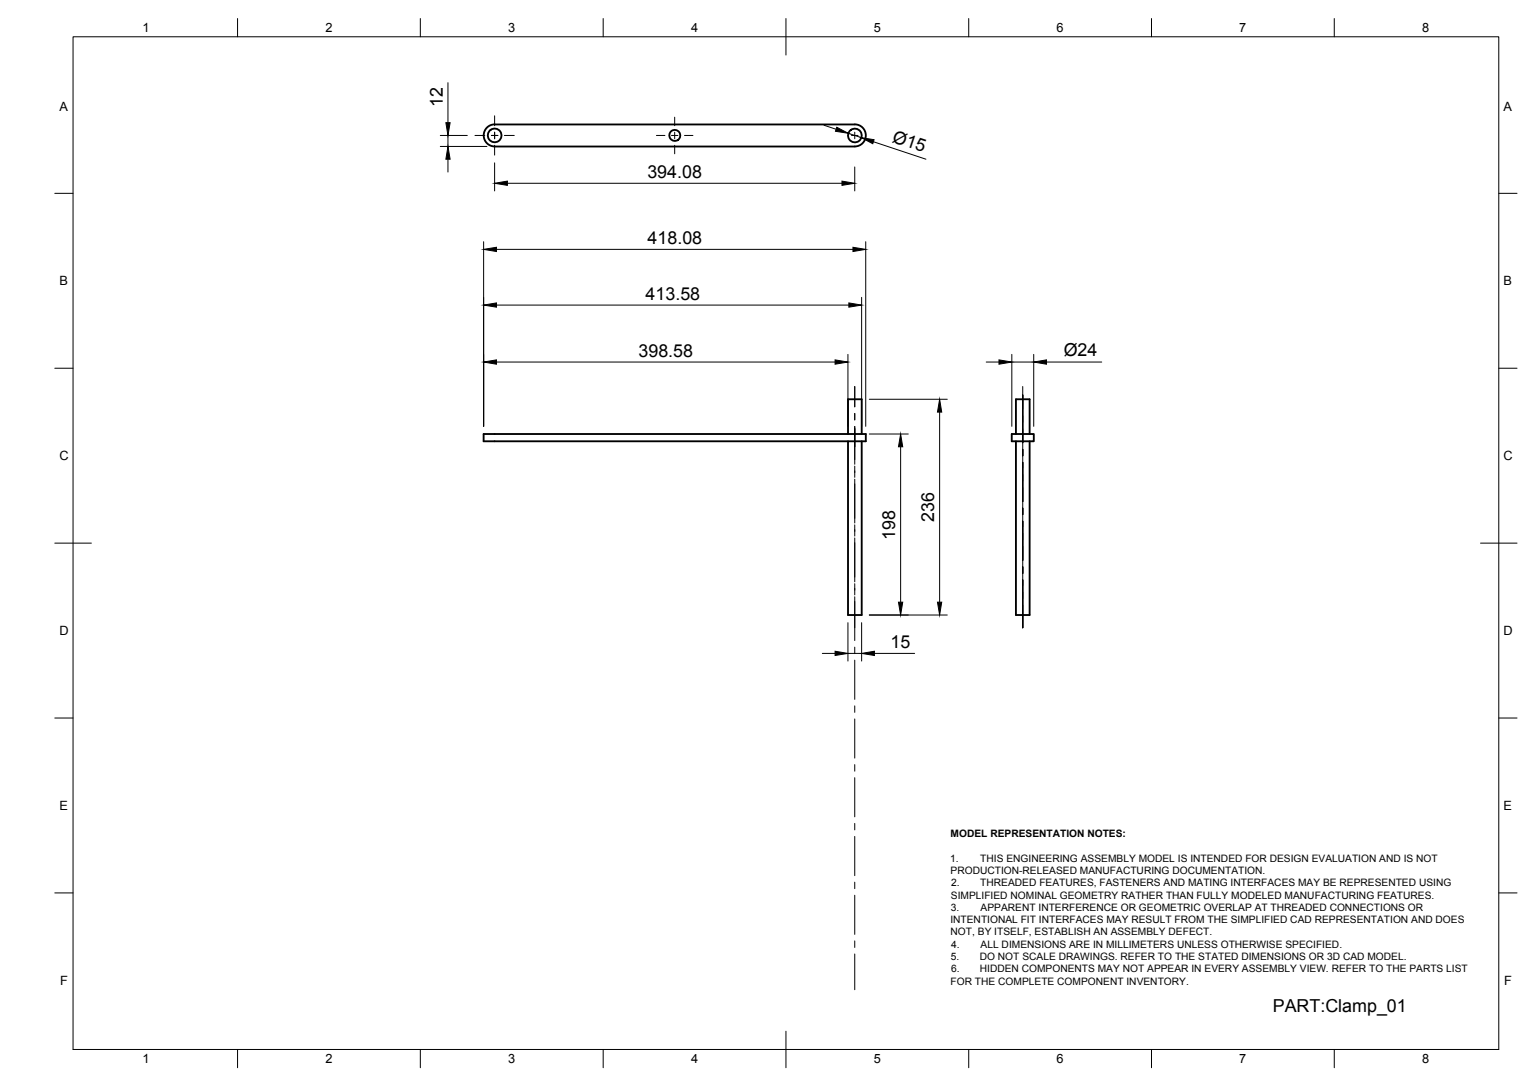
ISO-10303-21;
HEADER;
/* Generated by software containing ST-Developer
 * from STEP Tools, Inc. (www.steptools.com) 
 */

FILE_DESCRIPTION(
/* description */ (''),
/* implementation_level */ '2;1');

FILE_NAME(
/* name */ 'Clamp_01.step',
/* time_stamp */ '2026-10-05T15:35:09-07:00',
/* author */ (''),
/* organization */ (''),
/* preprocessor_version */ 'ST-DEVELOPER v20.2',
/* originating_system */ 'Autodesk Translation Framework v15.15.0.0',
/* authorisation */ '');

FILE_SCHEMA (('AUTOMOTIVE_DESIGN { 1 0 10303 214 3 1 1 }'));
ENDSEC;

DATA;
#10=MECHANICAL_DESIGN_GEOMETRIC_PRESENTATION_REPRESENTATION('',(#546),#74523);
#528=SHAPE_REPRESENTATION_RELATIONSHIP('SRR','None',#74561,#537);
#537=ADVANCED_BREP_SHAPE_REPRESENTATION('',(#555),#74517);
#546=STYLED_ITEM('',(#74612),#555);
#555=MANIFOLD_SOLID_BREP('Body1',#4725);
#581=FACE_BOUND('',#905,.T.);
#582=FACE_BOUND('',#906,.T.);
#583=FACE_BOUND('',#907,.T.);
#584=FACE_BOUND('',#909,.T.);
#585=FACE_BOUND('',#910,.T.);
#586=FACE_BOUND('',#911,.T.);
#637=PLANE('',#4942);
#638=PLANE('',#4946);
#639=PLANE('',#4950);
#640=PLANE('',#4952);
#641=PLANE('',#4956);
#642=PLANE('',#4959);
#734=FACE_OUTER_BOUND('',#898,.T.);
#735=FACE_OUTER_BOUND('',#899,.T.);
#736=FACE_OUTER_BOUND('',#900,.T.);
#737=FACE_OUTER_BOUND('',#901,.T.);
#738=FACE_OUTER_BOUND('',#902,.T.);
#739=FACE_OUTER_BOUND('',#903,.T.);
#740=FACE_OUTER_BOUND('',#904,.T.);
#741=FACE_OUTER_BOUND('',#908,.T.);
#742=FACE_OUTER_BOUND('',#912,.T.);
#743=FACE_OUTER_BOUND('',#913,.T.);
#744=FACE_OUTER_BOUND('',#914,.T.);
#745=FACE_OUTER_BOUND('',#915,.T.);
#898=EDGE_LOOP('',(#3222,#3223,#3224,#3225));
#899=EDGE_LOOP('',(#3226,#3227,#3228,#3229));
#900=EDGE_LOOP('',(#3230,#3231,#3232,#3233));
#901=EDGE_LOOP('',(#3234,#3235,#3236,#3237));
#902=EDGE_LOOP('',(#3238,#3239,#3240,#3241));
#903=EDGE_LOOP('',(#3242,#3243,#3244,#3245));
#904=EDGE_LOOP('',(#3246,#3247,#3248,#3249));
#905=EDGE_LOOP('',(#3250));
#906=EDGE_LOOP('',(#3251));
#907=EDGE_LOOP('',(#3252));
#908=EDGE_LOOP('',(#3253,#3254,#3255,#3256));
#909=EDGE_LOOP('',(#3257));
#910=EDGE_LOOP('',(#3258));
#911=EDGE_LOOP('',(#3259));
#912=EDGE_LOOP('',(#3260,#3261,#3262,#3263));
#913=EDGE_LOOP('',(#3264));
#914=EDGE_LOOP('',(#3265,#3266,#3267,#3268));
#915=EDGE_LOOP('',(#3269));
#1102=LINE('',#6110,#1299);
#1103=LINE('',#6116,#1300);
#1104=LINE('',#6121,#1301);
#1105=LINE('',#6123,#1302);
#1106=LINE('',#6125,#1303);
#1107=LINE('',#6126,#1304);
#1108=LINE('',#6131,#1305);
#1109=LINE('',#6135,#1306);
#1110=LINE('',#6137,#1307);
#1111=LINE('',#6138,#1308);
#1112=LINE('',#6151,#1309);
#1113=LINE('',#6156,#1310);
#1299=VECTOR('',#5396,6.00000000000001);
#1300=VECTOR('',#5403,7.5);
#1301=VECTOR('',#5408,10.);
#1302=VECTOR('',#5409,10.);
#1303=VECTOR('',#5410,10.);
#1304=VECTOR('',#5411,10.);
#1305=VECTOR('',#5416,10.);
#1306=VECTOR('',#5421,10.);
#1307=VECTOR('',#5422,10.);
#1308=VECTOR('',#5423,10.);
#1309=VECTOR('',#5442,7.5);
#1310=VECTOR('',#5449,7.5);
#1460=CIRCLE('',#4937,6.00000000000001);
#1461=CIRCLE('',#4938,6.00000000000001);
#1462=CIRCLE('',#4940,7.5);
#1463=CIRCLE('',#4941,7.5);
#1464=CIRCLE('',#4944,12.);
#1465=CIRCLE('',#4945,12.);
#1466=CIRCLE('',#4948,12.);
#1467=CIRCLE('',#4949,12.);
#1468=CIRCLE('',#4951,7.5);
#1469=CIRCLE('',#4953,7.5);
#1470=CIRCLE('',#4955,7.5);
#1471=CIRCLE('',#4957,7.5);
#1610=VERTEX_POINT('',#6107);
#1611=VERTEX_POINT('',#6109);
#1612=VERTEX_POINT('',#6113);
#1613=VERTEX_POINT('',#6115);
#1614=VERTEX_POINT('',#6119);
#1615=VERTEX_POINT('',#6120);
#1616=VERTEX_POINT('',#6122);
#1617=VERTEX_POINT('',#6124);
#1618=VERTEX_POINT('',#6128);
#1619=VERTEX_POINT('',#6130);
#1620=VERTEX_POINT('',#6134);
#1621=VERTEX_POINT('',#6136);
#1622=VERTEX_POINT('',#6143);
#1623=VERTEX_POINT('',#6146);
#1624=VERTEX_POINT('',#6149);
#1625=VERTEX_POINT('',#6153);
#2312=EDGE_CURVE('',#1610,#1610,#1460,.T.);
#2313=EDGE_CURVE('',#1610,#1611,#1102,.T.);
#2314=EDGE_CURVE('',#1611,#1611,#1461,.T.);
#2315=EDGE_CURVE('',#1612,#1612,#1462,.T.);
#2316=EDGE_CURVE('',#1612,#1613,#1103,.T.);
#2317=EDGE_CURVE('',#1613,#1613,#1463,.T.);
#2318=EDGE_CURVE('',#1614,#1615,#1104,.T.);
#2319=EDGE_CURVE('',#1614,#1616,#1105,.T.);
#2320=EDGE_CURVE('',#1616,#1617,#1106,.T.);
#2321=EDGE_CURVE('',#1615,#1617,#1107,.T.);
#2322=EDGE_CURVE('',#1618,#1614,#1464,.T.);
#2323=EDGE_CURVE('',#1618,#1619,#1108,.T.);
#2324=EDGE_CURVE('',#1619,#1616,#1465,.T.);
#2325=EDGE_CURVE('',#1620,#1618,#1109,.T.);
#2326=EDGE_CURVE('',#1620,#1621,#1110,.T.);
#2327=EDGE_CURVE('',#1621,#1619,#1111,.T.);
#2328=EDGE_CURVE('',#1615,#1620,#1466,.T.);
#2329=EDGE_CURVE('',#1617,#1621,#1467,.T.);
#2330=EDGE_CURVE('',#1622,#1622,#1468,.T.);
#2331=EDGE_CURVE('',#1623,#1623,#1469,.T.);
#2332=EDGE_CURVE('',#1624,#1624,#1470,.T.);
#2333=EDGE_CURVE('',#1624,#1623,#1112,.T.);
#2334=EDGE_CURVE('',#1625,#1625,#1471,.T.);
#2335=EDGE_CURVE('',#1622,#1625,#1113,.T.);
#3222=ORIENTED_EDGE('',*,*,#2312,.F.);
#3223=ORIENTED_EDGE('',*,*,#2313,.T.);
#3224=ORIENTED_EDGE('',*,*,#2314,.F.);
#3225=ORIENTED_EDGE('',*,*,#2313,.F.);
#3226=ORIENTED_EDGE('',*,*,#2315,.T.);
#3227=ORIENTED_EDGE('',*,*,#2316,.T.);
#3228=ORIENTED_EDGE('',*,*,#2317,.F.);
#3229=ORIENTED_EDGE('',*,*,#2316,.F.);
#3230=ORIENTED_EDGE('',*,*,#2318,.F.);
#3231=ORIENTED_EDGE('',*,*,#2319,.T.);
#3232=ORIENTED_EDGE('',*,*,#2320,.T.);
#3233=ORIENTED_EDGE('',*,*,#2321,.F.);
#3234=ORIENTED_EDGE('',*,*,#2322,.F.);
#3235=ORIENTED_EDGE('',*,*,#2323,.T.);
#3236=ORIENTED_EDGE('',*,*,#2324,.T.);
#3237=ORIENTED_EDGE('',*,*,#2319,.F.);
#3238=ORIENTED_EDGE('',*,*,#2325,.F.);
#3239=ORIENTED_EDGE('',*,*,#2326,.T.);
#3240=ORIENTED_EDGE('',*,*,#2327,.T.);
#3241=ORIENTED_EDGE('',*,*,#2323,.F.);
#3242=ORIENTED_EDGE('',*,*,#2328,.F.);
#3243=ORIENTED_EDGE('',*,*,#2321,.T.);
#3244=ORIENTED_EDGE('',*,*,#2329,.T.);
#3245=ORIENTED_EDGE('',*,*,#2326,.F.);
#3246=ORIENTED_EDGE('',*,*,#2329,.F.);
#3247=ORIENTED_EDGE('',*,*,#2320,.F.);
#3248=ORIENTED_EDGE('',*,*,#2324,.F.);
#3249=ORIENTED_EDGE('',*,*,#2327,.F.);
#3250=ORIENTED_EDGE('',*,*,#2312,.T.);
#3251=ORIENTED_EDGE('',*,*,#2315,.F.);
#3252=ORIENTED_EDGE('',*,*,#2330,.F.);
#3253=ORIENTED_EDGE('',*,*,#2328,.T.);
#3254=ORIENTED_EDGE('',*,*,#2325,.T.);
#3255=ORIENTED_EDGE('',*,*,#2322,.T.);
#3256=ORIENTED_EDGE('',*,*,#2318,.T.);
#3257=ORIENTED_EDGE('',*,*,#2314,.T.);
#3258=ORIENTED_EDGE('',*,*,#2317,.T.);
#3259=ORIENTED_EDGE('',*,*,#2331,.F.);
#3260=ORIENTED_EDGE('',*,*,#2332,.F.);
#3261=ORIENTED_EDGE('',*,*,#2333,.T.);
#3262=ORIENTED_EDGE('',*,*,#2331,.T.);
#3263=ORIENTED_EDGE('',*,*,#2333,.F.);
#3264=ORIENTED_EDGE('',*,*,#2334,.T.);
#3265=ORIENTED_EDGE('',*,*,#2330,.T.);
#3266=ORIENTED_EDGE('',*,*,#2335,.T.);
#3267=ORIENTED_EDGE('',*,*,#2334,.F.);
#3268=ORIENTED_EDGE('',*,*,#2335,.F.);
#3269=ORIENTED_EDGE('',*,*,#2332,.T.);
#4538=CYLINDRICAL_SURFACE('',#4936,6.00000000000001);
#4539=CYLINDRICAL_SURFACE('',#4939,7.5);
#4540=CYLINDRICAL_SURFACE('',#4943,12.);
#4541=CYLINDRICAL_SURFACE('',#4947,12.);
#4542=CYLINDRICAL_SURFACE('',#4954,7.5);
#4543=CYLINDRICAL_SURFACE('',#4958,7.5);
#4630=ADVANCED_FACE('',(#734),#4538,.F.);
#4631=ADVANCED_FACE('',(#735),#4539,.F.);
#4632=ADVANCED_FACE('',(#736),#637,.F.);
#4633=ADVANCED_FACE('',(#737),#4540,.T.);
#4634=ADVANCED_FACE('',(#738),#638,.F.);
#4635=ADVANCED_FACE('',(#739),#4541,.T.);
#4636=ADVANCED_FACE('',(#740,#581,#582,#583),#639,.F.);
#4637=ADVANCED_FACE('',(#741,#584,#585,#586),#640,.T.);
#4638=ADVANCED_FACE('',(#742),#4542,.T.);
#4639=ADVANCED_FACE('',(#743),#641,.F.);
#4640=ADVANCED_FACE('',(#744),#4543,.T.);
#4641=ADVANCED_FACE('',(#745),#642,.T.);
#4725=CLOSED_SHELL('',(#4630,#4631,#4632,#4633,#4634,#4635,#4636,#4637,
#4638,#4639,#4640,#4641));
#4935=AXIS2_PLACEMENT_3D('',#6105,#5390,#5391);
#4936=AXIS2_PLACEMENT_3D('',#6106,#5392,#5393);
#4937=AXIS2_PLACEMENT_3D('',#6108,#5394,#5395);
#4938=AXIS2_PLACEMENT_3D('',#6111,#5397,#5398);
#4939=AXIS2_PLACEMENT_3D('',#6112,#5399,#5400);
#4940=AXIS2_PLACEMENT_3D('',#6114,#5401,#5402);
#4941=AXIS2_PLACEMENT_3D('',#6117,#5404,#5405);
#4942=AXIS2_PLACEMENT_3D('',#6118,#5406,#5407);
#4943=AXIS2_PLACEMENT_3D('',#6127,#5412,#5413);
#4944=AXIS2_PLACEMENT_3D('',#6129,#5414,#5415);
#4945=AXIS2_PLACEMENT_3D('',#6132,#5417,#5418);
#4946=AXIS2_PLACEMENT_3D('',#6133,#5419,#5420);
#4947=AXIS2_PLACEMENT_3D('',#6139,#5424,#5425);
#4948=AXIS2_PLACEMENT_3D('',#6140,#5426,#5427);
#4949=AXIS2_PLACEMENT_3D('',#6141,#5428,#5429);
#4950=AXIS2_PLACEMENT_3D('',#6142,#5430,#5431);
#4951=AXIS2_PLACEMENT_3D('',#6144,#5432,#5433);
#4952=AXIS2_PLACEMENT_3D('',#6145,#5434,#5435);
#4953=AXIS2_PLACEMENT_3D('',#6147,#5436,#5437);
#4954=AXIS2_PLACEMENT_3D('',#6148,#5438,#5439);
#4955=AXIS2_PLACEMENT_3D('',#6150,#5440,#5441);
#4956=AXIS2_PLACEMENT_3D('',#6152,#5443,#5444);
#4957=AXIS2_PLACEMENT_3D('',#6154,#5445,#5446);
#4958=AXIS2_PLACEMENT_3D('',#6155,#5447,#5448);
#4959=AXIS2_PLACEMENT_3D('',#6157,#5450,#5451);
#5390=DIRECTION('axis',(0.,0.,1.));
#5391=DIRECTION('refdir',(1.,0.,0.));
#5392=DIRECTION('center_axis',(0.,1.,0.));
#5393=DIRECTION('ref_axis',(1.,0.,0.));
#5394=DIRECTION('center_axis',(0.,1.,0.));
#5395=DIRECTION('ref_axis',(1.,0.,0.));
#5396=DIRECTION('',(0.,1.,0.));
#5397=DIRECTION('center_axis',(0.,-1.,0.));
#5398=DIRECTION('ref_axis',(1.,0.,0.));
#5399=DIRECTION('center_axis',(0.,1.,0.));
#5400=DIRECTION('ref_axis',(1.,0.,0.));
#5401=DIRECTION('center_axis',(0.,-1.,0.));
#5402=DIRECTION('ref_axis',(1.,0.,0.));
#5403=DIRECTION('',(0.,1.,0.));
#5404=DIRECTION('center_axis',(0.,-1.,0.));
#5405=DIRECTION('ref_axis',(1.,0.,0.));
#5406=DIRECTION('center_axis',(0.812015371342714,0.,-0.583636048152575));
#5407=DIRECTION('ref_axis',(0.583636048152575,0.,0.812015371342714));
#5408=DIRECTION('',(0.583636048152575,0.,0.812015371342714));
#5409=DIRECTION('',(0.,-1.,0.));
#5410=DIRECTION('',(0.583636048152575,0.,0.812015371342714));
#5411=DIRECTION('',(0.,-1.,0.));
#5412=DIRECTION('center_axis',(0.,1.,0.));
#5413=DIRECTION('ref_axis',(0.812015371342714,0.,-0.583636048152574));
#5414=DIRECTION('center_axis',(0.,1.,0.));
#5415=DIRECTION('ref_axis',(0.812015371342714,0.,-0.583636048152574));
#5416=DIRECTION('',(0.,-1.,0.));
#5417=DIRECTION('center_axis',(0.,1.,0.));
#5418=DIRECTION('ref_axis',(0.812015371342714,0.,-0.583636048152574));
#5419=DIRECTION('center_axis',(-0.812015371342714,0.,0.583636048152575));
#5420=DIRECTION('ref_axis',(-0.583636048152575,0.,-0.812015371342714));
#5421=DIRECTION('',(-0.583636048152575,0.,-0.812015371342714));
#5422=DIRECTION('',(0.,-1.,0.));
#5423=DIRECTION('',(-0.583636048152575,0.,-0.812015371342714));
#5424=DIRECTION('center_axis',(0.,1.,0.));
#5425=DIRECTION('ref_axis',(-0.812015371342714,0.,0.583636048152574));
#5426=DIRECTION('center_axis',(0.,1.,0.));
#5427=DIRECTION('ref_axis',(-0.812015371342714,0.,0.583636048152574));
#5428=DIRECTION('center_axis',(0.,1.,0.));
#5429=DIRECTION('ref_axis',(-0.812015371342714,0.,0.583636048152574));
#5430=DIRECTION('center_axis',(0.,1.,0.));
#5431=DIRECTION('ref_axis',(1.,0.,0.));
#5432=DIRECTION('center_axis',(0.,-1.,0.));
#5433=DIRECTION('ref_axis',(1.,0.,0.));
#5434=DIRECTION('center_axis',(0.,1.,0.));
#5435=DIRECTION('ref_axis',(1.,0.,0.));
#5436=DIRECTION('center_axis',(0.,1.,0.));
#5437=DIRECTION('ref_axis',(1.,0.,0.));
#5438=DIRECTION('center_axis',(0.,1.,0.));
#5439=DIRECTION('ref_axis',(1.,0.,0.));
#5440=DIRECTION('center_axis',(0.,1.,0.));
#5441=DIRECTION('ref_axis',(1.,0.,0.));
#5442=DIRECTION('',(0.,-1.,0.));
#5443=DIRECTION('center_axis',(0.,1.,0.));
#5444=DIRECTION('ref_axis',(1.,0.,0.));
#5445=DIRECTION('center_axis',(0.,-1.,0.));
#5446=DIRECTION('ref_axis',(1.,0.,0.));
#5447=DIRECTION('center_axis',(0.,1.,0.));
#5448=DIRECTION('ref_axis',(1.,0.,0.));
#5449=DIRECTION('',(0.,-1.,0.));
#5450=DIRECTION('center_axis',(0.,1.,0.));
#5451=DIRECTION('ref_axis',(1.,0.,0.));
#6105=CARTESIAN_POINT('',(0.,0.,0.));
#6106=CARTESIAN_POINT('Origin',(60.231676812499,95.,175.));
#6107=CARTESIAN_POINT('',(54.231676812499,72.,175.));
#6108=CARTESIAN_POINT('Origin',(60.231676812499,72.,175.));
#6109=CARTESIAN_POINT('',(54.231676812499,80.,175.));
#6110=CARTESIAN_POINT('',(54.231676812499,95.,175.));
#6111=CARTESIAN_POINT('Origin',(60.231676812499,80.,175.));
#6112=CARTESIAN_POINT('Origin',(175.231676812499,80.,335.));
#6113=CARTESIAN_POINT('',(167.731676812499,72.,335.));
#6114=CARTESIAN_POINT('Origin',(175.231676812499,72.,335.));
#6115=CARTESIAN_POINT('',(167.731676812499,80.,335.));
#6116=CARTESIAN_POINT('',(167.731676812499,80.,335.));
#6117=CARTESIAN_POINT('Origin',(175.231676812499,80.,335.));
#6118=CARTESIAN_POINT('Origin',(-64.5125076436135,80.,22.0036325778309));
#6119=CARTESIAN_POINT('',(-64.5125076436135,80.,22.0036325778309));
#6120=CARTESIAN_POINT('',(165.487492356386,80.,342.003632577831));
#6121=CARTESIAN_POINT('',(-64.5125076436135,80.,22.0036325778309));
#6122=CARTESIAN_POINT('',(-64.5125076436135,72.,22.0036325778309));
#6123=CARTESIAN_POINT('',(-64.5125076436135,80.,22.0036325778309));
#6124=CARTESIAN_POINT('',(165.487492356386,72.,342.003632577831));
#6125=CARTESIAN_POINT('',(-64.5125076436135,72.,22.0036325778309));
#6126=CARTESIAN_POINT('',(165.487492356386,80.,342.003632577831));
#6127=CARTESIAN_POINT('Origin',(-54.7683231875009,80.,15.));
#6128=CARTESIAN_POINT('',(-45.0241387313884,80.,7.99636742216912));
#6129=CARTESIAN_POINT('Origin',(-54.7683231875009,80.,15.));
#6130=CARTESIAN_POINT('',(-45.0241387313884,72.,7.99636742216912));
#6131=CARTESIAN_POINT('',(-45.0241387313884,80.,7.99636742216912));
#6132=CARTESIAN_POINT('Origin',(-54.7683231875009,72.,15.));
#6133=CARTESIAN_POINT('Origin',(184.975861268612,80.,327.996367422169));
#6134=CARTESIAN_POINT('',(184.975861268612,80.,327.996367422169));
#6135=CARTESIAN_POINT('',(184.975861268612,80.,327.996367422169));
#6136=CARTESIAN_POINT('',(184.975861268612,72.,327.996367422169));
#6137=CARTESIAN_POINT('',(184.975861268612,80.,327.996367422169));
#6138=CARTESIAN_POINT('',(184.975861268612,72.,327.996367422169));
#6139=CARTESIAN_POINT('Origin',(175.231676812499,80.,335.));
#6140=CARTESIAN_POINT('Origin',(175.231676812499,80.,335.));
#6141=CARTESIAN_POINT('Origin',(175.231676812499,72.,335.));
#6142=CARTESIAN_POINT('Origin',(60.231676812499,72.,175.));
#6143=CARTESIAN_POINT('',(-62.2683231875009,72.,15.));
#6144=CARTESIAN_POINT('Origin',(-54.7683231875009,72.,15.));
#6145=CARTESIAN_POINT('Origin',(60.231676812499,80.,175.));
#6146=CARTESIAN_POINT('',(-62.2683231875009,80.,15.));
#6147=CARTESIAN_POINT('Origin',(-54.7683231875009,80.,15.));
#6148=CARTESIAN_POINT('Origin',(-54.7683231875009,0.,15.));
#6149=CARTESIAN_POINT('',(-62.2683231875009,118.,15.));
#6150=CARTESIAN_POINT('Origin',(-54.7683231875009,118.,15.));
#6151=CARTESIAN_POINT('',(-62.2683231875009,0.,15.));
#6152=CARTESIAN_POINT('Origin',(-54.7683231875009,-118.,15.));
#6153=CARTESIAN_POINT('',(-62.2683231875009,-118.,15.));
#6154=CARTESIAN_POINT('Origin',(-54.7683231875009,-118.,15.));
#6155=CARTESIAN_POINT('Origin',(-54.7683231875009,0.,15.));
#6156=CARTESIAN_POINT('',(-62.2683231875009,0.,15.));
#6157=CARTESIAN_POINT('Origin',(-54.7683231875009,118.,15.));
#74506=UNCERTAINTY_MEASURE_WITH_UNIT(LENGTH_MEASURE(0.01),#74524,
'DISTANCE_ACCURACY_VALUE',
'Maximum model space distance between geometric entities at asserted c
onnectivities');
#74512=UNCERTAINTY_MEASURE_WITH_UNIT(LENGTH_MEASURE(0.01),#74524,
'DISTANCE_ACCURACY_VALUE',
'Maximum model space distance between geometric entities at asserted c
onnectivities');
#74517=(
GEOMETRIC_REPRESENTATION_CONTEXT(3)
GLOBAL_UNCERTAINTY_ASSIGNED_CONTEXT((#74506))
GLOBAL_UNIT_ASSIGNED_CONTEXT((#74524,#74526,#74527))
REPRESENTATION_CONTEXT('','3D')
);
#74523=(
GEOMETRIC_REPRESENTATION_CONTEXT(3)
GLOBAL_UNCERTAINTY_ASSIGNED_CONTEXT((#74512))
GLOBAL_UNIT_ASSIGNED_CONTEXT((#74524,#74526,#74527))
REPRESENTATION_CONTEXT('','3D')
);
#74524=(
LENGTH_UNIT()
NAMED_UNIT(*)
SI_UNIT(.MILLI.,.METRE.)
);
#74526=(
NAMED_UNIT(*)
PLANE_ANGLE_UNIT()
SI_UNIT($,.RADIAN.)
);
#74527=(
NAMED_UNIT(*)
SI_UNIT($,.STERADIAN.)
SOLID_ANGLE_UNIT()
);
#74532=SHAPE_DEFINITION_REPRESENTATION(#74542,#74561);
#74542=PRODUCT_DEFINITION_SHAPE('',$,#74572);
#74561=SHAPE_REPRESENTATION('',(#4935),#74517);
#74567=PRODUCT_DEFINITION_CONTEXT('part definition',#74599,'design');
#74572=PRODUCT_DEFINITION('Clamp_01','Clamp_01',#74582,#74567);
#74582=PRODUCT_DEFINITION_FORMATION('',$,#74605);
#74599=APPLICATION_CONTEXT(
'Core Data for Automotive Mechanical Design Process');
#74600=PRODUCT_CONTEXT('part definition',#74599,'mechanical');
#74605=PRODUCT('Clamp_01','Clamp_01',$,(#74600));
#74612=PRESENTATION_STYLE_ASSIGNMENT((#74615));
#74615=SURFACE_STYLE_USAGE(.BOTH.,#74618);
#74618=SURFACE_SIDE_STYLE('',(#74621));
#74621=SURFACE_STYLE_FILL_AREA(#74624);
#74624=FILL_AREA_STYLE('Opaque(215,0,0)',(#74627));
#74627=FILL_AREA_STYLE_COLOUR('Opaque(215,0,0)',#74630);
#74630=COLOUR_RGB('Opaque(215,0,0)', 0.09019608, 0.27058824, 0.51372549);
ENDSEC;
END-ISO-10303-21;
